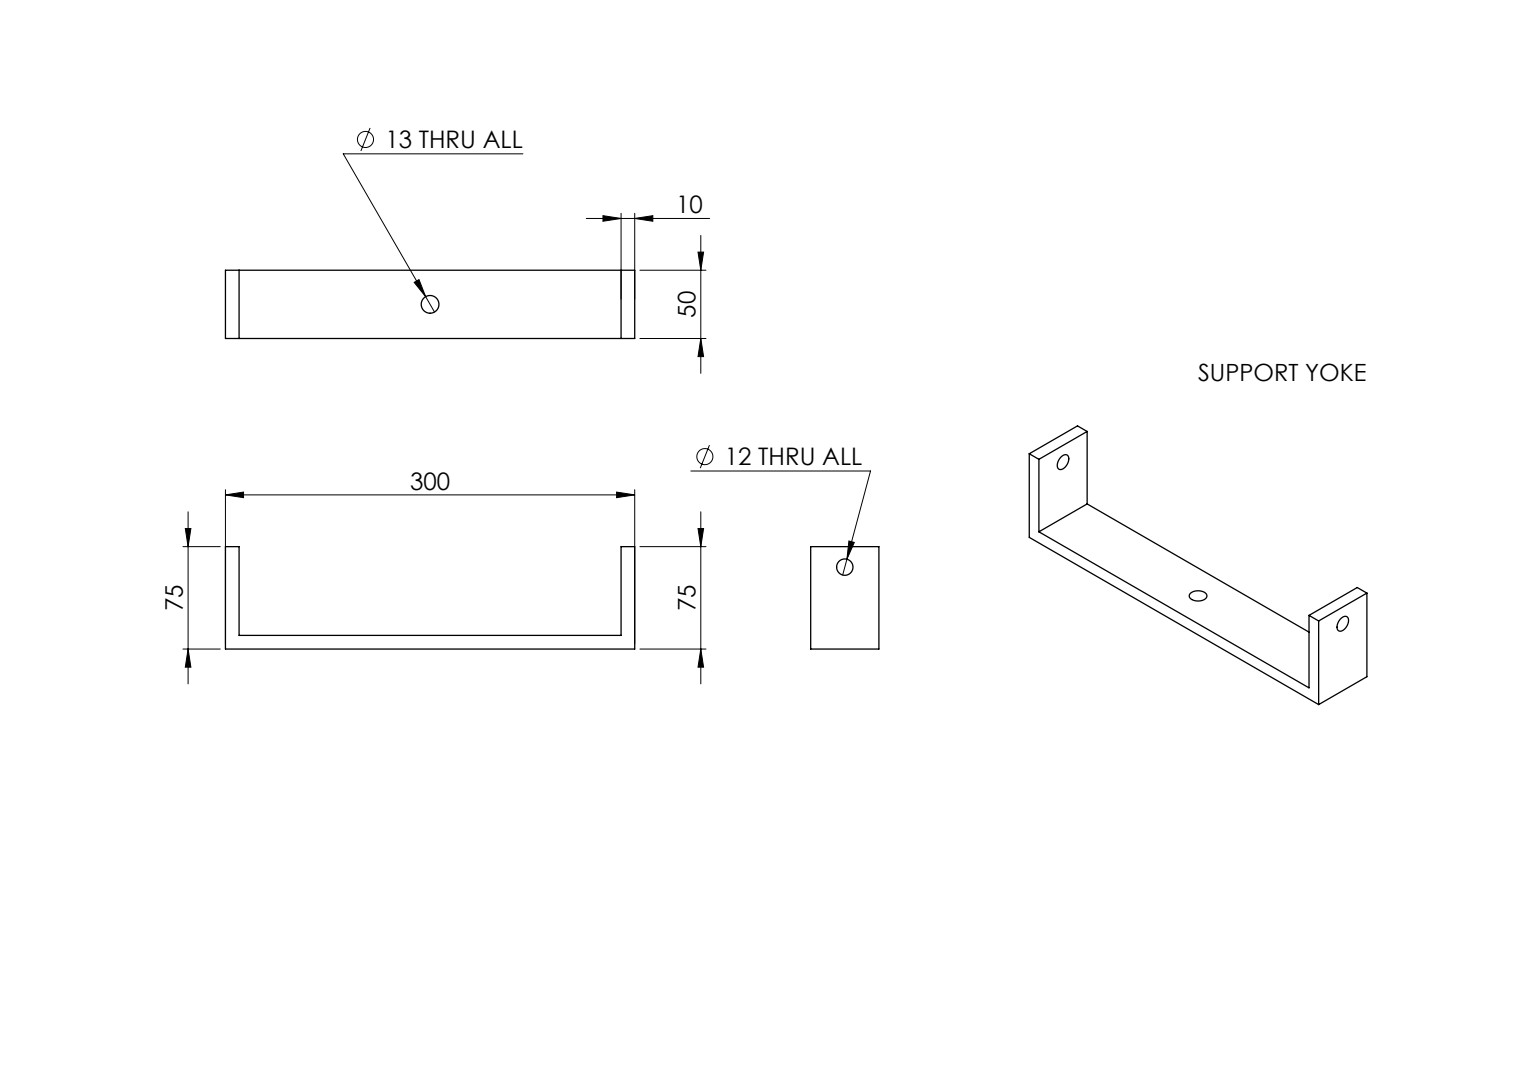
ISO-10303-21;
HEADER;
FILE_DESCRIPTION (('STEP AP214'),
    '1' );
FILE_NAME ('support yoke.step',
    '2026-10-22T16:49:52',
    ( '' ),
    ( '' ),
    'SwSTEP 2.0',
    'SolidWorks 2026',
    '' );
FILE_SCHEMA (( 'AUTOMOTIVE_DESIGN' ));
ENDSEC;

DATA;
#7=DIRECTION ( 'NONE',  ( 0.000000000000000000, 0.000000000000000000, -1.000000000000000000 ) ) ;
#8=DIRECTION ( 'NONE',  ( -1.000000000000000000, -0.000000000000000000, -0.000000000000000000 ) ) ;
#20=EDGE_LOOP ( 'NONE', ( #1630, #2560 ) ) ;
#23=ORIENTED_EDGE ( 'NONE', *, *, #198, .T. ) ;
#30=CARTESIAN_POINT ( 'NONE',  ( 150.0000000000000000, 810.0000000000000000, 25.00000000000000000 ) ) ;
#33=EDGE_LOOP ( 'NONE', ( #4983, #5227 ) ) ;
#50=CARTESIAN_POINT ( 'NONE',  ( -150.0000000000000000, 870.0000000000000000, 0.000000000000000000 ) ) ;
#67=STYLED_ITEM('',(#5412),#3780);
#72=CARTESIAN_POINT ( 'NONE',  ( -150.0000000000000000, 820.0000000000001137, 25.00000000000000000 ) ) ;
#79=EDGE_CURVE ( 'NONE', #3280, #3385, #2552, .T. ) ;
#80=EDGE_CURVE ( 'NONE', #4039, #3851, #2630, .T. ) ;
#99=ORIENTED_EDGE ( 'NONE', *, *, #4103, .T. ) ;
#103=DIRECTION ( 'NONE',  ( 1.000000000000000000, 0.000000000000000000, 0.000000000000000000 ) ) ;
#106=DIRECTION ( 'NONE',  ( 1.000000000000000000, 0.000000000000000000, 0.000000000000000000 ) ) ;
#112=PLANE ( 'NONE',  #5289 ) ;
#116=VECTOR ( 'NONE', #4178, 1000.000000000000000 ) ;
#148=VECTOR ( 'NONE', #4543, 1000.000000000000000 ) ;
#160=ORIENTED_EDGE ( 'NONE', *, *, #3298, .F. ) ;
#162=CARTESIAN_POINT ( 'NONE',  ( -150.0000000000000000, 870.0000000000000000, -6.000000000000006217 ) ) ;
#165=VERTEX_POINT ( 'NONE', #2690 ) ;
#191=DIRECTION ( 'NONE',  ( -0.000000000000000000, -1.000000000000000000, 0.000000000000000000 ) ) ;
#192=DIRECTION ( 'NONE',  ( -0.000000000000000000, 1.000000000000000000, -0.000000000000000000 ) ) ;
#197=ORIENTED_EDGE ( 'NONE', *, *, #3520, .F. ) ;
#198=EDGE_CURVE ( 'NONE', #3942, #4623, #5254, .T. ) ;
#206=EDGE_CURVE ( 'NONE', #3842, #5043, #2268, .T. ) ;
#238=ORIENTED_EDGE ( 'NONE', *, *, #1651, .F. ) ;
#247=CARTESIAN_POINT ( 'NONE',  ( 139.9999999999999716, 885.0000000000000000, -25.00000000000000000 ) ) ;
#249=ORIENTED_EDGE ( 'NONE', *, *, #342, .F. ) ;
#262=DIRECTION ( 'NONE',  ( 1.000000000000000000, 0.000000000000000000, 0.000000000000000000 ) ) ;
#280=CARTESIAN_POINT ( 'NONE',  ( 139.9999999999999716, 885.0000000000000000, 25.00000000000000000 ) ) ;
#286=EDGE_LOOP ( 'NONE', ( #1725, #726, #2392, #4939 ) ) ;
#300=VECTOR ( 'NONE', #2784, 1000.000000000000000 ) ;
#305=ADVANCED_FACE ( 'NONE', ( #1215, #3776 ), #1663, .T. ) ;
#330=DIRECTION ( 'NONE',  ( 0.000000000000000000, 0.000000000000000000, 1.000000000000000000 ) ) ;
#336=CIRCLE ( 'NONE', #2605, 5.999999999999894307 ) ;
#342=EDGE_CURVE ( 'NONE', #2324, #5253, #4160, .T. ) ;
#351=ORIENTED_EDGE ( 'NONE', *, *, #3520, .T. ) ;
#359=DIRECTION ( 'NONE',  ( 0.000000000000000000, 0.000000000000000000, -1.000000000000000000 ) ) ;
#371=DIRECTION ( 'NONE',  ( -0.000000000000000000, -0.000000000000000000, -1.000000000000000000 ) ) ;
#374=ORIENTED_EDGE ( 'NONE', *, *, #3449, .T. ) ;
#376=CARTESIAN_POINT ( 'NONE',  ( 139.9999999999999716, 820.0000000000001137, -25.00000000000000000 ) ) ;
#397=ORIENTED_EDGE ( 'NONE', *, *, #4687, .F. ) ;
#413=DIRECTION ( 'NONE',  ( 0.000000000000000000, 0.000000000000000000, 1.000000000000000000 ) ) ;
#427=ORIENTED_EDGE ( 'NONE', *, *, #4247, .F. ) ;
#436=CARTESIAN_POINT ( 'NONE',  ( -150.0000000000000000, 870.0000000000000000, -5.999999999999950262 ) ) ;
#443=PRODUCT ( 'support yoke', 'support yoke', '', ( #4465 ) ) ;
#451=ORIENTED_EDGE ( 'NONE', *, *, #2561, .F. ) ;
#455=ORIENTED_EDGE ( 'NONE', *, *, #4975, .F. ) ;
#457=VERTEX_POINT ( 'NONE', #162 ) ;
#485=( GEOMETRIC_REPRESENTATION_CONTEXT ( 3 ) GLOBAL_UNCERTAINTY_ASSIGNED_CONTEXT ( ( #3762 ) ) GLOBAL_UNIT_ASSIGNED_CONTEXT ( ( #4296, #3410, #1343 ) ) REPRESENTATION_CONTEXT ( 'NONE', 'WORKASPACE' ) );
#486=EDGE_LOOP ( 'NONE', ( #2087, #1135, #1675, #1922 ) ) ;
#489=DIRECTION ( 'NONE',  ( 1.000000000000000000, 0.000000000000000000, 0.000000000000000000 ) ) ;
#503=VERTEX_POINT ( 'NONE', #879 ) ;
#509=CIRCLE ( 'NONE', #2248, 6.499999999999999112 ) ;
#530=VECTOR ( 'NONE', #4346, 1000.000000000000000 ) ;
#535=EDGE_CURVE ( 'NONE', #4624, #5043, #1720, .T. ) ;
#556=PRESENTATION_STYLE_ASSIGNMENT (( #4250 ) ) ;
#570=CARTESIAN_POINT ( 'NONE',  ( -150.0000000000000000, 810.0000000000000000, -25.00000000000000000 ) ) ;
#583=CARTESIAN_POINT ( 'NONE',  ( 7.960204194457795477E-16, 810.0000000000000000, -6.499999999999999112 ) ) ;
#584=VECTOR ( 'NONE', #1682, 1000.000000000000000 ) ;
#586=LINE ( 'NONE', #5193, #5037 ) ;
#653=COLOUR_RGB ( '',0.8941176470588234615, 0.8941176470588234615, 0.8941176470588234615 ) ;
#654=ORIENTED_EDGE ( 'NONE', *, *, #80, .T. ) ;
#677=CARTESIAN_POINT ( 'NONE',  ( -150.0000000000000000, 810.0000000000000000, 25.00000000000000000 ) ) ;
#686=CARTESIAN_POINT ( 'NONE',  ( 150.0000000000000000, 885.0000000000000000, -25.00000000000000000 ) ) ;
#699=DIRECTION ( 'NONE',  ( 0.000000000000000000, 0.000000000000000000, 1.000000000000000000 ) ) ;
#705=ORIENTED_EDGE ( 'NONE', *, *, #198, .F. ) ;
#726=ORIENTED_EDGE ( 'NONE', *, *, #1041, .T. ) ;
#732=ORIENTED_EDGE ( 'NONE', *, *, #3637, .T. ) ;
#739=DIRECTION ( 'NONE',  ( 1.000000000000000000, -0.000000000000000000, -0.000000000000000000 ) ) ;
#766=DIRECTION ( 'NONE',  ( 0.000000000000000000, 0.000000000000000000, 1.000000000000000000 ) ) ;
#768=( GEOMETRIC_REPRESENTATION_CONTEXT ( 3 ) GLOBAL_UNCERTAINTY_ASSIGNED_CONTEXT ( ( #2886 ) ) GLOBAL_UNIT_ASSIGNED_CONTEXT ( ( #2204, #5209, #5150 ) ) REPRESENTATION_CONTEXT ( 'NONE', 'WORKASPACE' ) );
#769=DIRECTION ( 'NONE',  ( 1.000000000000000000, 0.000000000000000000, 0.000000000000000000 ) ) ;
#786=CARTESIAN_POINT ( 'NONE',  ( 139.9999999999999716, 885.0000000000000000, -25.00000000000000000 ) ) ;
#788=APPLICATION_CONTEXT ( 'automotive_design' ) ;
#800=LINE ( 'NONE', #247, #2779 ) ;
#814=EDGE_CURVE ( 'NONE', #3015, #3385, #852, .T. ) ;
#820=ORIENTED_EDGE ( 'NONE', *, *, #3637, .F. ) ;
#831=DIRECTION ( 'NONE',  ( -1.000000000000000000, 0.000000000000000000, 0.000000000000000000 ) ) ;
#836=CIRCLE ( 'NONE', #1178, 6.000000000000005329 ) ;
#837=ORIENTED_EDGE ( 'NONE', *, *, #4975, .T. ) ;
#843=CYLINDRICAL_SURFACE ( 'NONE', #2403, 6.500000000000000000 ) ;
#844=ORIENTED_EDGE ( 'NONE', *, *, #814, .F. ) ;
#849=VECTOR ( 'NONE', #191, 1000.000000000000000 ) ;
#850=VERTEX_POINT ( 'NONE', #5295 ) ;
#852=LINE ( 'NONE', #2846, #116 ) ;
#873=FACE_BOUND ( 'NONE', #4726, .T. ) ;
#875=ADVANCED_FACE ( 'NONE', ( #4126 ), #1205, .T. ) ;
#876=EDGE_CURVE ( 'NONE', #3385, #3280, #4904, .T. ) ;
#878=ORIENTED_EDGE ( 'NONE', *, *, #3994, .T. ) ;
#879=CARTESIAN_POINT ( 'NONE',  ( -150.0000000000000000, 810.0000000000000000, 25.00000000000000000 ) ) ;
#883=ORIENTED_EDGE ( 'NONE', *, *, #876, .F. ) ;
#891=DIRECTION ( 'NONE',  ( 0.000000000000000000, 0.000000000000000000, -1.000000000000000000 ) ) ;
#906=VECTOR ( 'NONE', #371, 1000.000000000000000 ) ;
#921=CIRCLE ( 'NONE', #2511, 5.999999999999894307 ) ;
#928=VECTOR ( 'NONE', #4600, 1000.000000000000000 ) ;
#950=DIRECTION ( 'NONE',  ( -1.000000000000000000, -0.000000000000000000, 0.000000000000000000 ) ) ;
#954=ORIENTED_EDGE ( 'NONE', *, *, #3467, .T. ) ;
#990=FILL_AREA_STYLE_COLOUR ( '', #653 ) ;
#992=EDGE_CURVE ( 'NONE', #1518, #3842, #1759, .T. ) ;
#998=AXIS2_PLACEMENT_3D ( 'NONE', #1508, #1083, #4072 ) ;
#1011=AXIS2_PLACEMENT_3D ( 'NONE', #2490, #2911, #4155 ) ;
#1017=LINE ( 'NONE', #4706, #2766 ) ;
#1027=ORIENTED_EDGE ( 'NONE', *, *, #2170, .F. ) ;
#1030=AXIS2_PLACEMENT_3D ( 'NONE', #4574, #3774, #413 ) ;
#1041=EDGE_CURVE ( 'NONE', #3303, #457, #1786, .T. ) ;
#1053=VECTOR ( 'NONE', #5134, 1000.000000000000000 ) ;
#1083=DIRECTION ( 'NONE',  ( 0.000000000000000000, 1.000000000000000000, 0.000000000000000000 ) ) ;
#1086=ORIENTED_EDGE ( 'NONE', *, *, #4012, .F. ) ;
#1098=DIRECTION ( 'NONE',  ( 0.000000000000000000, 0.000000000000000000, -1.000000000000000000 ) ) ;
#1102=EDGE_CURVE ( 'NONE', #4507, #850, #2281, .T. ) ;
#1108=ORIENTED_EDGE ( 'NONE', *, *, #79, .F. ) ;
#1127=CARTESIAN_POINT ( 'NONE',  ( 0.000000000000000000, 0.000000000000000000, 25.00000000000000000 ) ) ;
#1135=ORIENTED_EDGE ( 'NONE', *, *, #5039, .F. ) ;
#1137=EDGE_LOOP ( 'NONE', ( #2340, #4405, #654, #2970 ) ) ;
#1145=CARTESIAN_POINT ( 'NONE',  ( -139.9999999999999716, 810.0000000000000000, 25.00000000000000000 ) ) ;
#1155=CARTESIAN_POINT ( 'NONE',  ( -150.0000000000000000, 870.0000000000000000, 0.000000000000000000 ) ) ;
#1174=DIRECTION ( 'NONE',  ( 1.000000000000000000, 0.000000000000000000, -0.000000000000000000 ) ) ;
#1175=DIRECTION ( 'NONE',  ( 0.000000000000000000, 0.000000000000000000, 1.000000000000000000 ) ) ;
#1178=AXIS2_PLACEMENT_3D ( 'NONE', #50, #2614, #2635 ) ;
#1192=LINE ( 'NONE', #4977, #3207 ) ;
#1205=PLANE ( 'NONE',  #4466 ) ;
#1215=FACE_BOUND ( 'NONE', #3739, .T. ) ;
#1224=VERTEX_POINT ( 'NONE', #3925 ) ;
#1233=PLANE ( 'NONE',  #1011 ) ;
#1243=DIRECTION ( 'NONE',  ( -0.000000000000000000, -0.000000000000000000, -1.000000000000000000 ) ) ;
#1248=EDGE_CURVE ( 'NONE', #503, #3980, #2343, .T. ) ;
#1266=STYLED_ITEM ( 'NONE', ( #556 ), #5266 ) ;
#1268=ORIENTED_EDGE ( 'NONE', *, *, #1102, .F. ) ;
#1271=DIRECTION ( 'NONE',  ( -0.000000000000000000, -1.000000000000000000, -0.000000000000000000 ) ) ;
#1292=EDGE_CURVE ( 'NONE', #165, #2065, #2179, .T. ) ;
#1304=PLANE ( 'NONE',  #3654 ) ;
#1316=CARTESIAN_POINT ( 'NONE',  ( -150.0000000000000000, 870.0000000000000000, 0.000000000000000000 ) ) ;
#1323=LINE ( 'NONE', #4743, #2686 ) ;
#1325=AXIS2_PLACEMENT_3D ( 'NONE', #3342, #2525, #5331 ) ;
#1343=( NAMED_UNIT ( * ) SI_UNIT ( $, .STERADIAN. ) SOLID_ANGLE_UNIT ( ) );
#1345=MECHANICAL_DESIGN_GEOMETRIC_PRESENTATION_REPRESENTATION('',(#1266),#5013);
#1357=ORIENTED_EDGE ( 'NONE', *, *, #4166, .F. ) ;
#1359=CARTESIAN_POINT ( 'NONE',  ( -139.9999999999999716, 870.0000000000000000, 5.999999999999950262 ) ) ;
#1375=CARTESIAN_POINT ( 'NONE',  ( -139.9999999999999716, 820.0000000000001137, -25.00000000000000000 ) ) ;
#1379=CARTESIAN_POINT ( 'NONE',  ( -150.0000000000000000, 820.0000000000001137, -25.00000000000000000 ) ) ;
#1423=AXIS2_PLACEMENT_3D ( 'NONE', #1316, #2995, #2132 ) ;
#1428=EDGE_LOOP ( 'NONE', ( #3649, #4159, #2102, #844 ) ) ;
#1438=CARTESIAN_POINT ( 'NONE',  ( 150.0000000000000000, 885.0000000000000000, 25.00000000000000000 ) ) ;
#1444=VECTOR ( 'NONE', #2559, 1000.000000000000000 ) ;
#1464=ORIENTED_EDGE ( 'NONE', *, *, #1248, .F. ) ;
#1487=DIRECTION ( 'NONE',  ( 1.000000000000000000, 0.000000000000000000, 0.000000000000000000 ) ) ;
#1495=CARTESIAN_POINT ( 'NONE',  ( -150.0000000000000000, 870.0000000000000000, 0.000000000000000000 ) ) ;
#1498=FACE_OUTER_BOUND ( 'NONE', #1428, .T. ) ;
#1508=CARTESIAN_POINT ( 'NONE',  ( -150.0000000000000000, 810.0000000000000000, 25.00000000000000000 ) ) ;
#1518=VERTEX_POINT ( 'NONE', #2242 ) ;
#1564=ORIENTED_EDGE ( 'NONE', *, *, #2240, .T. ) ;
#1565=ORIENTED_EDGE ( 'NONE', *, *, #2151, .F. ) ;
#1577=LINE ( 'NONE', #4909, #4491 ) ;
#1584=EDGE_LOOP ( 'NONE', ( #1586, #820, #5321, #4418 ) ) ;
#1586=ORIENTED_EDGE ( 'NONE', *, *, #3467, .F. ) ;
#1595=ORIENTED_EDGE ( 'NONE', *, *, #2067, .F. ) ;
#1599=DIRECTION ( 'NONE',  ( 0.000000000000000000, 0.000000000000000000, 1.000000000000000000 ) ) ;
#1607=PRODUCT_DEFINITION_CONTEXT ( 'detailed design', #4664, 'design' ) ;
#1614=ORIENTED_EDGE ( 'NONE', *, *, #1292, .T. ) ;
#1620=SHAPE_REPRESENTATION ( 'support yoke', ( #4154 ), #485 ) ;
#1630=ORIENTED_EDGE ( 'NONE', *, *, #5039, .T. ) ;
#1635=FACE_OUTER_BOUND ( 'NONE', #1658, .T. ) ;
#1645=CARTESIAN_POINT ( 'NONE',  ( 150.0000000000000000, 810.0000000000000000, 25.00000000000000000 ) ) ;
#1651=EDGE_CURVE ( 'NONE', #3303, #3154, #3622, .T. ) ;
#1658=EDGE_LOOP ( 'NONE', ( #3325, #1595, #1614, #732 ) ) ;
#1663=PLANE ( 'NONE',  #1325 ) ;
#1675=ORIENTED_EDGE ( 'NONE', *, *, #814, .T. ) ;
#1682=DIRECTION ( 'NONE',  ( 0.000000000000000000, 1.000000000000000000, 0.000000000000000000 ) ) ;
#1707=CIRCLE ( 'NONE', #1423, 6.000000000000005329 ) ;
#1712=ORIENTED_EDGE ( 'NONE', *, *, #3751, .T. ) ;
#1720=LINE ( 'NONE', #5048, #4511 ) ;
#1725=ORIENTED_EDGE ( 'NONE', *, *, #3298, .T. ) ;
#1735=EDGE_LOOP ( 'NONE', ( #2336, #2444, #4389, #3297 ) ) ;
#1748=PLANE ( 'NONE',  #2875 ) ;
#1757=ORIENTED_EDGE ( 'NONE', *, *, #206, .T. ) ;
#1759=LINE ( 'NONE', #4692, #3954 ) ;
#1773=CARTESIAN_POINT ( 'NONE',  ( 139.9999999999999716, 885.0000000000000000, 25.00000000000000000 ) ) ;
#1779=ORIENTED_EDGE ( 'NONE', *, *, #4990, .F. ) ;
#1783=ORIENTED_EDGE ( 'NONE', *, *, #535, .F. ) ;
#1786=LINE ( 'NONE', #2093, #5353 ) ;
#1805=DIRECTION ( 'NONE',  ( -1.000000000000000000, -0.000000000000000000, 0.000000000000000000 ) ) ;
#1809=AXIS2_PLACEMENT_3D ( 'NONE', #3644, #4934, #1599 ) ;
#1822=CARTESIAN_POINT ( 'NONE',  ( -150.0000000000000000, 870.0000000000000000, 5.999999999999950262 ) ) ;
#1867=ORIENTED_EDGE ( 'NONE', *, *, #2240, .F. ) ;
#1882=LINE ( 'NONE', #2739, #4659 ) ;
#1922=ORIENTED_EDGE ( 'NONE', *, *, #876, .T. ) ;
#1925=CARTESIAN_POINT ( 'NONE',  ( -139.9999999999999716, 870.0000000000000000, 0.000000000000000000 ) ) ;
#1944=PLANE ( 'NONE',  #998 ) ;
#1945=AXIS2_PLACEMENT_3D ( 'NONE', #3613, #5271, #359 ) ;
#1953=CYLINDRICAL_SURFACE ( 'NONE', #1809, 5.999999999999950262 ) ;
#2015=DIRECTION ( 'NONE',  ( -1.000000000000000000, -0.000000000000000000, -0.000000000000000000 ) ) ;
#2024=EDGE_LOOP ( 'NONE', ( #1779, #5378, #5038, #249 ) ) ;
#2036=VERTEX_POINT ( 'NONE', #3689 ) ;
#2040=CYLINDRICAL_SURFACE ( 'NONE', #1030, 6.500000000000000000 ) ;
#2056=ADVANCED_FACE ( 'NONE', ( #2840 ), #843, .F. ) ;
#2065=VERTEX_POINT ( 'NONE', #2432 ) ;
#2067=EDGE_CURVE ( 'NONE', #165, #2036, #4515, .T. ) ;
#2070=ORIENTED_EDGE ( 'NONE', *, *, #2170, .T. ) ;
#2074=VECTOR ( 'NONE', #3618, 1000.000000000000000 ) ;
#2087=ORIENTED_EDGE ( 'NONE', *, *, #3943, .F. ) ;
#2088=ORIENTED_EDGE ( 'NONE', *, *, #1292, .F. ) ;
#2093=CARTESIAN_POINT ( 'NONE',  ( -150.0000000000000000, 870.0000000000000000, -5.999999999999950262 ) ) ;
#2102=ORIENTED_EDGE ( 'NONE', *, *, #79, .T. ) ;
#2126=FACE_OUTER_BOUND ( 'NONE', #1735, .T. ) ;
#2132=DIRECTION ( 'NONE',  ( 0.000000000000000000, 0.000000000000000000, 1.000000000000000000 ) ) ;
#2133=LINE ( 'NONE', #5002, #1444 ) ;
#2140=CARTESIAN_POINT ( 'NONE',  ( -150.0000000000000000, 810.0000000000000000, 25.00000000000000000 ) ) ;
#2142=CIRCLE ( 'NONE', #2860, 5.999999999999950262 ) ;
#2151=EDGE_CURVE ( 'NONE', #457, #3895, #836, .T. ) ;
#2170=EDGE_CURVE ( 'NONE', #165, #503, #3892, .T. ) ;
#2179=LINE ( 'NONE', #5123, #3715 ) ;
#2202=EDGE_LOOP ( 'NONE', ( #1268, #451, #4763, #1564 ) ) ;
#2204=( LENGTH_UNIT ( ) NAMED_UNIT ( * ) SI_UNIT ( .MILLI., .METRE. ) );
#2219=VECTOR ( 'NONE', #1271, 1000.000000000000000 ) ;
#2221=CIRCLE ( 'NONE', #2587, 6.499999999999999112 ) ;
#2228=CARTESIAN_POINT ( 'NONE',  ( -150.0000000000000000, 810.0000000000000000, -25.00000000000000000 ) ) ;
#2232=ORIENTED_EDGE ( 'NONE', *, *, #5241, .F. ) ;
#2240=EDGE_CURVE ( 'NONE', #5253, #850, #5182, .T. ) ;
#2242=CARTESIAN_POINT ( 'NONE',  ( 139.9999999999999716, 885.0000000000000000, 25.00000000000000000 ) ) ;
#2247=ORIENTED_EDGE ( 'NONE', *, *, #2067, .T. ) ;
#2248=AXIS2_PLACEMENT_3D ( 'NONE', #3992, #3161, #1175 ) ;
#2268=LINE ( 'NONE', #1438, #3844 ) ;
#2281=LINE ( 'NONE', #4377, #300 ) ;
#2296=LINE ( 'NONE', #3090, #849 ) ;
#2324=VERTEX_POINT ( 'NONE', #3507 ) ;
#2327=ADVANCED_FACE ( 'NONE', ( #1498 ), #3173, .F. ) ;
#2336=ORIENTED_EDGE ( 'NONE', *, *, #535, .T. ) ;
#2337=VECTOR ( 'NONE', #3898, 1000.000000000000000 ) ;
#2340=ORIENTED_EDGE ( 'NONE', *, *, #3767, .F. ) ;
#2343=LINE ( 'NONE', #677, #3085 ) ;
#2344=FACE_BOUND ( 'NONE', #33, .T. ) ;
#2386=LINE ( 'NONE', #280, #2074 ) ;
#2392=ORIENTED_EDGE ( 'NONE', *, *, #2151, .T. ) ;
#2403=AXIS2_PLACEMENT_3D ( 'NONE', #4485, #5343, #766 ) ;
#2405=CARTESIAN_POINT ( 'NONE',  ( 0.000000000000000000, 0.000000000000000000, -25.00000000000000000 ) ) ;
#2407=DIRECTION ( 'NONE',  ( 0.000000000000000000, 0.000000000000000000, -1.000000000000000000 ) ) ;
#2432=CARTESIAN_POINT ( 'NONE',  ( -139.9999999999999716, 885.0000000000000000, 25.00000000000000000 ) ) ;
#2434=CARTESIAN_POINT ( 'NONE',  ( 0.000000000000000000, 0.000000000000000000, 0.000000000000000000 ) ) ;
#2444=ORIENTED_EDGE ( 'NONE', *, *, #206, .F. ) ;
#2446=PLANE ( 'NONE',  #5377 ) ;
#2452=ORIENTED_EDGE ( 'NONE', *, *, #2562, .T. ) ;
#2455=CARTESIAN_POINT ( 'NONE',  ( -150.0000000000000000, 885.0000000000000000, 25.00000000000000000 ) ) ;
#2466=SHAPE_DEFINITION_REPRESENTATION ( #5021, #1620 ) ;
#2474=ORIENTED_EDGE ( 'NONE', *, *, #1651, .T. ) ;
#2489=FACE_OUTER_BOUND ( 'NONE', #5079, .T. ) ;
#2490=CARTESIAN_POINT ( 'NONE',  ( -150.0000000000000000, 885.0000000000000000, 25.00000000000000000 ) ) ;
#2511=AXIS2_PLACEMENT_3D ( 'NONE', #3251, #2015, #3226 ) ;
#2525=DIRECTION ( 'NONE',  ( 0.000000000000000000, 1.000000000000000000, 0.000000000000000000 ) ) ;
#2552=CIRCLE ( 'NONE', #2988, 5.999999999999950262 ) ;
#2558=CARTESIAN_POINT ( 'NONE',  ( 0.000000000000000000, 810.0000000000000000, 0.000000000000000000 ) ) ;
#2559=DIRECTION ( 'NONE',  ( -0.000000000000000000, -0.000000000000000000, -1.000000000000000000 ) ) ;
#2560=ORIENTED_EDGE ( 'NONE', *, *, #3359, .T. ) ;
#2561=EDGE_CURVE ( 'NONE', #2324, #4507, #2221, .T. ) ;
#2562=EDGE_CURVE ( 'NONE', #3895, #457, #1707, .T. ) ;
#2587=AXIS2_PLACEMENT_3D ( 'NONE', #2558, #4211, #2632 ) ;
#2605=AXIS2_PLACEMENT_3D ( 'NONE', #4464, #5350, #4414 ) ;
#2614=DIRECTION ( 'NONE',  ( -1.000000000000000000, -0.000000000000000000, -0.000000000000000000 ) ) ;
#2626=PLANE ( 'NONE',  #3396 ) ;
#2630=LINE ( 'NONE', #72, #1053 ) ;
#2632=DIRECTION ( 'NONE',  ( 0.000000000000000000, 0.000000000000000000, 1.000000000000000000 ) ) ;
#2635=DIRECTION ( 'NONE',  ( 0.000000000000000000, 0.000000000000000000, 1.000000000000000000 ) ) ;
#2637=EDGE_CURVE ( 'NONE', #850, #5253, #5278, .T. ) ;
#2666=SURFACE_STYLE_FILL_AREA ( #3509 ) ;
#2686=VECTOR ( 'NONE', #4009, 1000.000000000000000 ) ;
#2690=CARTESIAN_POINT ( 'NONE',  ( -150.0000000000000000, 885.0000000000000000, 25.00000000000000000 ) ) ;
#2699=SURFACE_SIDE_STYLE ('',( #2666 ) ) ;
#2724=ORIENTED_EDGE ( 'NONE', *, *, #1248, .T. ) ;
#2736=AXIS2_PLACEMENT_3D ( 'NONE', #3726, #4078, #330 ) ;
#2739=CARTESIAN_POINT ( 'NONE',  ( -150.0000000000000000, 810.0000000000000000, -25.00000000000000000 ) ) ;
#2745=CARTESIAN_POINT ( 'NONE',  ( -139.9999999999999716, 820.0000000000001137, 25.00000000000000000 ) ) ;
#2766=VECTOR ( 'NONE', #4317, 1000.000000000000000 ) ;
#2772=DIRECTION ( 'NONE',  ( -1.000000000000000000, -0.000000000000000000, -0.000000000000000000 ) ) ;
#2775=ADVANCED_FACE ( 'NONE', ( #3170 ), #4003, .F. ) ;
#2777=CARTESIAN_POINT ( 'NONE',  ( -150.0000000000000000, 870.0000000000000000, 0.000000000000000000 ) ) ;
#2778=DIRECTION ( 'NONE',  ( -0.000000000000000000, -1.000000000000000000, 0.000000000000000000 ) ) ;
#2779=VECTOR ( 'NONE', #1487, 1000.000000000000000 ) ;
#2784=DIRECTION ( 'NONE',  ( -0.000000000000000000, 1.000000000000000000, -0.000000000000000000 ) ) ;
#2789=FACE_BOUND ( 'NONE', #4125, .T. ) ;
#2816=CARTESIAN_POINT ( 'NONE',  ( 150.0000000000000000, 885.0000000000000000, 25.00000000000000000 ) ) ;
#2822=FACE_OUTER_BOUND ( 'NONE', #4974, .T. ) ;
#2827=ORIENTED_EDGE ( 'NONE', *, *, #1041, .F. ) ;
#2840=FACE_OUTER_BOUND ( 'NONE', #2202, .T. ) ;
#2846=CARTESIAN_POINT ( 'NONE',  ( -150.0000000000000000, 870.0000000000000000, 5.999999999999950262 ) ) ;
#2857=DIRECTION ( 'NONE',  ( -0.000000000000000000, -0.000000000000000000, -1.000000000000000000 ) ) ;
#2860=AXIS2_PLACEMENT_3D ( 'NONE', #1925, #739, #2407 ) ;
#2875=AXIS2_PLACEMENT_3D ( 'NONE', #1645, #831, #3758 ) ;
#2882=DIRECTION ( 'NONE',  ( -1.000000000000000000, 0.000000000000000000, -0.000000000000000000 ) ) ;
#2886=UNCERTAINTY_MEASURE_WITH_UNIT (LENGTH_MEASURE( 1.000000000000000082E-05 ), #2204, 'distance_accuracy_value', 'NONE');
#2910=CARTESIAN_POINT ( 'NONE',  ( -139.9999999999999716, 820.0000000000001137, 25.00000000000000000 ) ) ;
#2911=DIRECTION ( 'NONE',  ( 0.000000000000000000, 1.000000000000000000, 0.000000000000000000 ) ) ;
#2922=ORIENTED_EDGE ( 'NONE', *, *, #3767, .T. ) ;
#2936=LINE ( 'NONE', #30, #584 ) ;
#2949=EDGE_LOOP ( 'NONE', ( #2827, #2474, #1712, #2452 ) ) ;
#2962=LINE ( 'NONE', #3394, #928 ) ;
#2970=ORIENTED_EDGE ( 'NONE', *, *, #4395, .T. ) ;
#2988=AXIS2_PLACEMENT_3D ( 'NONE', #2994, #1805, #3913 ) ;
#2994=CARTESIAN_POINT ( 'NONE',  ( 139.9999999999999716, 870.0000000000000000, 0.000000000000000000 ) ) ;
#2995=DIRECTION ( 'NONE',  ( -1.000000000000000000, -0.000000000000000000, -0.000000000000000000 ) ) ;
#3013=FACE_BOUND ( 'NONE', #20, .T. ) ;
#3015=VERTEX_POINT ( 'NONE', #3401 ) ;
#3023=( NAMED_UNIT ( * ) SI_UNIT ( $, .STERADIAN. ) SOLID_ANGLE_UNIT ( ) );
#3035=LINE ( 'NONE', #1822, #3108 ) ;
#3067=DIRECTION ( 'NONE',  ( 0.000000000000000000, 1.000000000000000000, 0.000000000000000000 ) ) ;
#3085=VECTOR ( 'NONE', #262, 1000.000000000000000 ) ;
#3090=CARTESIAN_POINT ( 'NONE',  ( -139.9999999999999716, 810.0000000000000000, -25.00000000000000000 ) ) ;
#3096=CLOSED_SHELL ( 'NONE', ( #5140, #2327, #2775, #4770, #3514, #4826, #305, #3388, #3411, #4018, #5385, #3597, #875, #5096, #4619, #2056 ) ) ;
#3108=VECTOR ( 'NONE', #4263, 1000.000000000000000 ) ;
#3134=LINE ( 'NONE', #2228, #2337 ) ;
#3143=ORIENTED_EDGE ( 'NONE', *, *, #80, .F. ) ;
#3152=ORIENTED_EDGE ( 'NONE', *, *, #2562, .F. ) ;
#3154=VERTEX_POINT ( 'NONE', #1359 ) ;
#3161=DIRECTION ( 'NONE',  ( -0.000000000000000000, 1.000000000000000000, -0.000000000000000000 ) ) ;
#3170=FACE_OUTER_BOUND ( 'NONE', #286, .T. ) ;
#3173=CYLINDRICAL_SURFACE ( 'NONE', #5095, 5.999999999999950262 ) ;
#3195=CARTESIAN_POINT ( 'NONE',  ( 139.9999999999999716, 870.0000000000000000, 5.999999999999950262 ) ) ;
#3203=DIRECTION ( 'NONE',  ( -1.000000000000000000, 0.000000000000000000, -0.000000000000000000 ) ) ;
#3207=VECTOR ( 'NONE', #1243, 1000.000000000000000 ) ;
#3226=DIRECTION ( 'NONE',  ( 0.000000000000000000, 0.000000000000000000, 1.000000000000000000 ) ) ;
#3251=CARTESIAN_POINT ( 'NONE',  ( 150.0000000000000000, 870.0000000000000000, 0.000000000000000000 ) ) ;
#3280=VERTEX_POINT ( 'NONE', #5325 ) ;
#3297=ORIENTED_EDGE ( 'NONE', *, *, #4012, .T. ) ;
#3298=EDGE_CURVE ( 'NONE', #3154, #3303, #2142, .T. ) ;
#3303=VERTEX_POINT ( 'NONE', #4080 ) ;
#3314=LINE ( 'NONE', #436, #4937 ) ;
#3325=ORIENTED_EDGE ( 'NONE', *, *, #4103, .F. ) ;
#3342=CARTESIAN_POINT ( 'NONE',  ( -150.0000000000000000, 820.0000000000001137, 25.00000000000000000 ) ) ;
#3348=EDGE_LOOP ( 'NONE', ( #455, #397, #4195, #1757 ) ) ;
#3359=EDGE_CURVE ( 'NONE', #1224, #3015, #921, .T. ) ;
#3362=LINE ( 'NONE', #2910, #148 ) ;
#3371=CARTESIAN_POINT ( 'NONE',  ( 0.000000000000000000, 820.0000000000001137, 6.500000000000000000 ) ) ;
#3385=VERTEX_POINT ( 'NONE', #3195 ) ;
#3388=ADVANCED_FACE ( 'NONE', ( #2789, #4047 ), #4874, .T. ) ;
#3394=CARTESIAN_POINT ( 'NONE',  ( 150.0000000000000000, 810.0000000000000000, 25.00000000000000000 ) ) ;
#3396=AXIS2_PLACEMENT_3D ( 'NONE', #4361, #950, #4284 ) ;
#3401=CARTESIAN_POINT ( 'NONE',  ( 150.0000000000000000, 870.0000000000000000, 5.999999999999894307 ) ) ;
#3410=( NAMED_UNIT ( * ) PLANE_ANGLE_UNIT ( ) SI_UNIT ( $, .RADIAN. ) );
#3411=ADVANCED_FACE ( 'NONE', ( #1635 ), #1233, .T. ) ;
#3449=EDGE_CURVE ( 'NONE', #2036, #3744, #1882, .T. ) ;
#3456=DIRECTION ( 'NONE',  ( 0.000000000000000000, -0.000000000000000000, 1.000000000000000000 ) ) ;
#3467=EDGE_CURVE ( 'NONE', #4833, #5330, #2296, .T. ) ;
#3507=CARTESIAN_POINT ( 'NONE',  ( 0.000000000000000000, 810.0000000000000000, 6.499999999999999112 ) ) ;
#3509=FILL_AREA_STYLE ('',( #990 ) ) ;
#3514=ADVANCED_FACE ( 'NONE', ( #4392 ), #112, .T. ) ;
#3520=EDGE_CURVE ( 'NONE', #3851, #1518, #1017, .T. ) ;
#3551=LINE ( 'NONE', #1379, #5384 ) ;
#3554=VECTOR ( 'NONE', #4468, 1000.000000000000000 ) ;
#3597=ADVANCED_FACE ( 'NONE', ( #2822 ), #2446, .F. ) ;
#3613=CARTESIAN_POINT ( 'NONE',  ( -139.9999999999999716, 870.0000000000000000, 0.000000000000000000 ) ) ;
#3618=DIRECTION ( 'NONE',  ( -0.000000000000000000, -0.000000000000000000, -1.000000000000000000 ) ) ;
#3622=CIRCLE ( 'NONE', #1945, 5.999999999999950262 ) ;
#3637=EDGE_CURVE ( 'NONE', #2065, #4833, #1577, .T. ) ;
#3644=CARTESIAN_POINT ( 'NONE',  ( -150.0000000000000000, 870.0000000000000000, 0.000000000000000000 ) ) ;
#3649=ORIENTED_EDGE ( 'NONE', *, *, #3359, .F. ) ;
#3654=AXIS2_PLACEMENT_3D ( 'NONE', #4620, #4153, #891 ) ;
#3689=CARTESIAN_POINT ( 'NONE',  ( -150.0000000000000000, 885.0000000000000000, -25.00000000000000000 ) ) ;
#3715=VECTOR ( 'NONE', #103, 1000.000000000000000 ) ;
#3726=CARTESIAN_POINT ( 'NONE',  ( 139.9999999999999716, 870.0000000000000000, 0.000000000000000000 ) ) ;
#3739=EDGE_LOOP ( 'NONE', ( #1867, #4810 ) ) ;
#3744=VERTEX_POINT ( 'NONE', #570 ) ;
#3751=EDGE_CURVE ( 'NONE', #3154, #3895, #3035, .T. ) ;
#3758=DIRECTION ( 'NONE',  ( 0.000000000000000000, 0.000000000000000000, 1.000000000000000000 ) ) ;
#3762=UNCERTAINTY_MEASURE_WITH_UNIT (LENGTH_MEASURE( 1.000000000000000082E-05 ), #4296, 'distance_accuracy_value', 'NONE');
#3767=EDGE_CURVE ( 'NONE', #5330, #3942, #3551, .T. ) ;
#3774=DIRECTION ( 'NONE',  ( -0.000000000000000000, 1.000000000000000000, -0.000000000000000000 ) ) ;
#3776=FACE_OUTER_BOUND ( 'NONE', #1137, .T. ) ;
#3780=MANIFOLD_SOLID_BREP ( 'M12 Clearance Hole1', #3096 ) ;
#3796=CARTESIAN_POINT ( 'NONE',  ( 150.0000000000000000, 810.0000000000000000, 25.00000000000000000 ) ) ;
#3800=AXIS2_PLACEMENT_3D ( 'NONE', #5163, #5192, #3973 ) ;
#3842=VERTEX_POINT ( 'NONE', #2816 ) ;
#3844=VECTOR ( 'NONE', #5217, 1000.000000000000000 ) ;
#3851=VERTEX_POINT ( 'NONE', #5262 ) ;
#3880=CARTESIAN_POINT ( 'NONE',  ( -139.9999999999999716, 885.0000000000000000, -25.00000000000000000 ) ) ;
#3892=LINE ( 'NONE', #2140, #2219 ) ;
#3895=VERTEX_POINT ( 'NONE', #4900 ) ;
#3898=DIRECTION ( 'NONE',  ( 1.000000000000000000, 0.000000000000000000, 0.000000000000000000 ) ) ;
#3911=ORIENTED_EDGE ( 'NONE', *, *, #4247, .T. ) ;
#3913=DIRECTION ( 'NONE',  ( 0.000000000000000000, 0.000000000000000000, 1.000000000000000000 ) ) ;
#3925=CARTESIAN_POINT ( 'NONE',  ( 150.0000000000000000, 870.0000000000000000, -5.999999999999894307 ) ) ;
#3939=DIRECTION ( 'NONE',  ( -0.000000000000000000, -1.000000000000000000, -0.000000000000000000 ) ) ;
#3942=VERTEX_POINT ( 'NONE', #376 ) ;
#3943=EDGE_CURVE ( 'NONE', #1224, #3280, #3314, .T. ) ;
#3954=VECTOR ( 'NONE', #489, 1000.000000000000000 ) ;
#3966=DIRECTION ( 'NONE',  ( 0.000000000000000000, 0.000000000000000000, 1.000000000000000000 ) ) ;
#3973=DIRECTION ( 'NONE',  ( 0.000000000000000000, 0.000000000000000000, 1.000000000000000000 ) ) ;
#3980=VERTEX_POINT ( 'NONE', #3796 ) ;
#3985=FACE_OUTER_BOUND ( 'NONE', #4365, .T. ) ;
#3992=CARTESIAN_POINT ( 'NONE',  ( 0.000000000000000000, 810.0000000000000000, 0.000000000000000000 ) ) ;
#3994=EDGE_CURVE ( 'NONE', #3980, #3842, #2936, .T. ) ;
#3999=EDGE_CURVE ( 'NONE', #4039, #5330, #3362, .T. ) ;
#4003=CYLINDRICAL_SURFACE ( 'NONE', #4323, 5.999999999999950262 ) ;
#4009=DIRECTION ( 'NONE',  ( 1.000000000000000000, 0.000000000000000000, 0.000000000000000000 ) ) ;
#4012=EDGE_CURVE ( 'NONE', #3980, #4624, #2962, .T. ) ;
#4018=ADVANCED_FACE ( 'NONE', ( #873, #2489 ), #1304, .F. ) ;
#4039=VERTEX_POINT ( 'NONE', #2745 ) ;
#4047=FACE_OUTER_BOUND ( 'NONE', #1584, .T. ) ;
#4048=FACE_OUTER_BOUND ( 'NONE', #2949, .T. ) ;
#4060=CYLINDRICAL_SURFACE ( 'NONE', #4666, 5.999999999999950262 ) ;
#4072=DIRECTION ( 'NONE',  ( 0.000000000000000000, -0.000000000000000000, 1.000000000000000000 ) ) ;
#4078=DIRECTION ( 'NONE',  ( -1.000000000000000000, -0.000000000000000000, 0.000000000000000000 ) ) ;
#4080=CARTESIAN_POINT ( 'NONE',  ( -139.9999999999999716, 870.0000000000000000, -5.999999999999950262 ) ) ;
#4103=EDGE_CURVE ( 'NONE', #2036, #4833, #1323, .T. ) ;
#4119=EDGE_LOOP ( 'NONE', ( #705, #4272, #351, #5336 ) ) ;
#4125=EDGE_LOOP ( 'NONE', ( #160, #238 ) ) ;
#4126=FACE_OUTER_BOUND ( 'NONE', #5128, .T. ) ;
#4153=DIRECTION ( 'NONE',  ( 1.000000000000000000, 0.000000000000000000, 0.000000000000000000 ) ) ;
#4154=AXIS2_PLACEMENT_3D ( 'NONE', #2434, #5290, #769 ) ;
#4155=DIRECTION ( 'NONE',  ( 0.000000000000000000, -0.000000000000000000, 1.000000000000000000 ) ) ;
#4159=ORIENTED_EDGE ( 'NONE', *, *, #3943, .T. ) ;
#4160=LINE ( 'NONE', #3371, #3554 ) ;
#4166=EDGE_CURVE ( 'NONE', #2065, #4039, #586, .T. ) ;
#4178=DIRECTION ( 'NONE',  ( -1.000000000000000000, -0.000000000000000000, -0.000000000000000000 ) ) ;
#4195=ORIENTED_EDGE ( 'NONE', *, *, #992, .T. ) ;
#4200=FACE_OUTER_BOUND ( 'NONE', #2024, .T. ) ;
#4211=DIRECTION ( 'NONE',  ( -0.000000000000000000, 1.000000000000000000, -0.000000000000000000 ) ) ;
#4247=EDGE_CURVE ( 'NONE', #503, #3744, #1192, .T. ) ;
#4250=SURFACE_STYLE_USAGE ( .BOTH. , #2699 ) ;
#4263=DIRECTION ( 'NONE',  ( -1.000000000000000000, -0.000000000000000000, -0.000000000000000000 ) ) ;
#4272=ORIENTED_EDGE ( 'NONE', *, *, #4395, .F. ) ;
#4284=DIRECTION ( 'NONE',  ( 0.000000000000000000, 0.000000000000000000, 1.000000000000000000 ) ) ;
#4296=( LENGTH_UNIT ( ) NAMED_UNIT ( * ) SI_UNIT ( .MILLI., .METRE. ) );
#4299=ORIENTED_EDGE ( 'NONE', *, *, #992, .F. ) ;
#4316=CARTESIAN_POINT ( 'NONE',  ( 139.9999999999999716, 810.0000000000000000, -25.00000000000000000 ) ) ;
#4317=DIRECTION ( 'NONE',  ( -0.000000000000000000, 1.000000000000000000, 0.000000000000000000 ) ) ;
#4318=PRODUCT_DEFINITION_FORMATION_WITH_SPECIFIED_SOURCE ( 'ANY', '', #443, .NOT_KNOWN. ) ;
#4321=AXIS2_PLACEMENT_3D ( 'NONE', #4348, #192, #3966 ) ;
#4323=AXIS2_PLACEMENT_3D ( 'NONE', #1495, #2772, #4823 ) ;
#4325=( LENGTH_UNIT ( ) NAMED_UNIT ( * ) SI_UNIT ( .MILLI., .METRE. ) );
#4346=DIRECTION ( 'NONE',  ( -0.000000000000000000, 1.000000000000000000, 0.000000000000000000 ) ) ;
#4348=CARTESIAN_POINT ( 'NONE',  ( 0.000000000000000000, 820.0000000000001137, 0.000000000000000000 ) ) ;
#4361=CARTESIAN_POINT ( 'NONE',  ( 139.9999999999999716, 810.0000000000000000, 25.00000000000000000 ) ) ;
#4365=EDGE_LOOP ( 'NONE', ( #4453, #1086, #1464, #3911 ) ) ;
#4377=CARTESIAN_POINT ( 'NONE',  ( 7.960204194457795477E-16, 820.0000000000001137, -6.500000000000000000 ) ) ;
#4389=ORIENTED_EDGE ( 'NONE', *, *, #3994, .F. ) ;
#4392=FACE_OUTER_BOUND ( 'NONE', #3348, .T. ) ;
#4395=EDGE_CURVE ( 'NONE', #3851, #3942, #2133, .T. ) ;
#4405=ORIENTED_EDGE ( 'NONE', *, *, #3999, .F. ) ;
#4414=DIRECTION ( 'NONE',  ( 0.000000000000000000, 0.000000000000000000, 1.000000000000000000 ) ) ;
#4418=ORIENTED_EDGE ( 'NONE', *, *, #3999, .T. ) ;
#4425=DIRECTION ( 'NONE',  ( -1.000000000000000000, -0.000000000000000000, -0.000000000000000000 ) ) ;
#4448=FACE_OUTER_BOUND ( 'NONE', #486, .T. ) ;
#4453=ORIENTED_EDGE ( 'NONE', *, *, #5241, .T. ) ;
#4464=CARTESIAN_POINT ( 'NONE',  ( 150.0000000000000000, 870.0000000000000000, 0.000000000000000000 ) ) ;
#4465=PRODUCT_CONTEXT ( 'NONE', #788, 'mechanical' ) ;
#4466=AXIS2_PLACEMENT_3D ( 'NONE', #2405, #7, #2882 ) ;
#4468=DIRECTION ( 'NONE',  ( -0.000000000000000000, 1.000000000000000000, -0.000000000000000000 ) ) ;
#4485=CARTESIAN_POINT ( 'NONE',  ( 0.000000000000000000, 820.0000000000001137, 0.000000000000000000 ) ) ;
#4491=VECTOR ( 'NONE', #2857, 1000.000000000000000 ) ;
#4507=VERTEX_POINT ( 'NONE', #583 ) ;
#4511=VECTOR ( 'NONE', #4625, 1000.000000000000000 ) ;
#4515=LINE ( 'NONE', #2455, #906 ) ;
#4543=DIRECTION ( 'NONE',  ( -0.000000000000000000, -0.000000000000000000, -1.000000000000000000 ) ) ;
#4574=CARTESIAN_POINT ( 'NONE',  ( 0.000000000000000000, 820.0000000000001137, 0.000000000000000000 ) ) ;
#4600=DIRECTION ( 'NONE',  ( -0.000000000000000000, -0.000000000000000000, -1.000000000000000000 ) ) ;
#4619=ADVANCED_FACE ( 'NONE', ( #4448 ), #4060, .F. ) ;
#4620=CARTESIAN_POINT ( 'NONE',  ( -150.0000000000000000, 810.0000000000000000, 25.00000000000000000 ) ) ;
#4623=VERTEX_POINT ( 'NONE', #786 ) ;
#4624=VERTEX_POINT ( 'NONE', #4943 ) ;
#4625=DIRECTION ( 'NONE',  ( 0.000000000000000000, 1.000000000000000000, 0.000000000000000000 ) ) ;
#4638=SHAPE_REPRESENTATION_RELATIONSHIP ( 'NONE' , 'NONE' ,  #1620, #5266 ) ;
#4659=VECTOR ( 'NONE', #3939, 1000.000000000000000 ) ;
#4661=UNCERTAINTY_MEASURE_WITH_UNIT (LENGTH_MEASURE( 1.000000000000000082E-05 ), #4325, 'distance_accuracy_value', 'NONE');
#4664=APPLICATION_CONTEXT ( 'automotive_design' ) ;
#4666=AXIS2_PLACEMENT_3D ( 'NONE', #1155, #4855, #5358 ) ;
#4667=( NAMED_UNIT ( * ) PLANE_ANGLE_UNIT ( ) SI_UNIT ( $, .RADIAN. ) );
#4670=DIRECTION ( 'NONE',  ( -1.000000000000000000, -0.000000000000000000, -0.000000000000000000 ) ) ;
#4687=EDGE_CURVE ( 'NONE', #1518, #4623, #2386, .T. ) ;
#4692=CARTESIAN_POINT ( 'NONE',  ( 139.9999999999999716, 885.0000000000000000, 25.00000000000000000 ) ) ;
#4706=CARTESIAN_POINT ( 'NONE',  ( 139.9999999999999716, 810.0000000000000000, 25.00000000000000000 ) ) ;
#4718=CARTESIAN_POINT ( 'NONE',  ( 0.000000000000000000, 820.0000000000001137, 6.500000000000000888 ) ) ;
#4726=EDGE_LOOP ( 'NONE', ( #3152, #1565 ) ) ;
#4727=FACE_BOUND ( 'NONE', #4870, .T. ) ;
#4743=CARTESIAN_POINT ( 'NONE',  ( -150.0000000000000000, 885.0000000000000000, -25.00000000000000000 ) ) ;
#4745=MECHANICAL_DESIGN_GEOMETRIC_PRESENTATION_REPRESENTATION('',(#67),#768);
#4763=ORIENTED_EDGE ( 'NONE', *, *, #342, .T. ) ;
#4770=ADVANCED_FACE ( 'NONE', ( #3013, #2126 ), #1748, .F. ) ;
#4788=FACE_OUTER_BOUND ( 'NONE', #4119, .T. ) ;
#4810=ORIENTED_EDGE ( 'NONE', *, *, #2637, .F. ) ;
#4823=DIRECTION ( 'NONE',  ( 0.000000000000000000, 0.000000000000000000, 1.000000000000000000 ) ) ;
#4826=ADVANCED_FACE ( 'NONE', ( #4727, #4788 ), #2626, .T. ) ;
#4833=VERTEX_POINT ( 'NONE', #3880 ) ;
#4855=DIRECTION ( 'NONE',  ( -1.000000000000000000, -0.000000000000000000, -0.000000000000000000 ) ) ;
#4870=EDGE_LOOP ( 'NONE', ( #883, #1108 ) ) ;
#4874=PLANE ( 'NONE',  #5191 ) ;
#4900=CARTESIAN_POINT ( 'NONE',  ( -150.0000000000000000, 870.0000000000000000, 6.000000000000005329 ) ) ;
#4904=CIRCLE ( 'NONE', #2736, 5.999999999999950262 ) ;
#4909=CARTESIAN_POINT ( 'NONE',  ( -139.9999999999999716, 885.0000000000000000, 25.00000000000000000 ) ) ;
#4925=ORIENTED_EDGE ( 'NONE', *, *, #3449, .F. ) ;
#4934=DIRECTION ( 'NONE',  ( -1.000000000000000000, -0.000000000000000000, -0.000000000000000000 ) ) ;
#4937=VECTOR ( 'NONE', #8, 1000.000000000000000 ) ;
#4939=ORIENTED_EDGE ( 'NONE', *, *, #3751, .F. ) ;
#4943=CARTESIAN_POINT ( 'NONE',  ( 150.0000000000000000, 810.0000000000000000, -25.00000000000000000 ) ) ;
#4974=EDGE_LOOP ( 'NONE', ( #878, #4299, #197, #3143, #1357, #2088, #2070, #2724 ) ) ;
#4975=EDGE_CURVE ( 'NONE', #4623, #5043, #800, .T. ) ;
#4977=CARTESIAN_POINT ( 'NONE',  ( -150.0000000000000000, 810.0000000000000000, 25.00000000000000000 ) ) ;
#4983=ORIENTED_EDGE ( 'NONE', *, *, #2561, .T. ) ;
#4990=EDGE_CURVE ( 'NONE', #4507, #2324, #509, .T. ) ;
#5002=CARTESIAN_POINT ( 'NONE',  ( 139.9999999999999716, 820.0000000000001137, 25.00000000000000000 ) ) ;
#5013=( GEOMETRIC_REPRESENTATION_CONTEXT ( 3 ) GLOBAL_UNCERTAINTY_ASSIGNED_CONTEXT ( ( #4661 ) ) GLOBAL_UNIT_ASSIGNED_CONTEXT ( ( #4325, #4667, #3023 ) ) REPRESENTATION_CONTEXT ( 'NONE', 'WORKASPACE' ) );
#5021=PRODUCT_DEFINITION_SHAPE ( 'NONE', 'NONE',  #5255 ) ;
#5037=VECTOR ( 'NONE', #2778, 1000.000000000000000 ) ;
#5038=ORIENTED_EDGE ( 'NONE', *, *, #2637, .T. ) ;
#5039=EDGE_CURVE ( 'NONE', #3015, #1224, #336, .T. ) ;
#5043=VERTEX_POINT ( 'NONE', #686 ) ;
#5048=CARTESIAN_POINT ( 'NONE',  ( 150.0000000000000000, 810.0000000000000000, -25.00000000000000000 ) ) ;
#5079=EDGE_LOOP ( 'NONE', ( #374, #427, #1027, #2247 ) ) ;
#5095=AXIS2_PLACEMENT_3D ( 'NONE', #2777, #4425, #699 ) ;
#5096=ADVANCED_FACE ( 'NONE', ( #4048 ), #1953, .F. ) ;
#5123=CARTESIAN_POINT ( 'NONE',  ( -150.0000000000000000, 885.0000000000000000, 25.00000000000000000 ) ) ;
#5128=EDGE_LOOP ( 'NONE', ( #1783, #2232, #4925, #99, #954, #2922, #23, #837 ) ) ;
#5134=DIRECTION ( 'NONE',  ( 1.000000000000000000, 0.000000000000000000, 0.000000000000000000 ) ) ;
#5140=ADVANCED_FACE ( 'NONE', ( #4200 ), #2040, .F. ) ;
#5150=( NAMED_UNIT ( * ) SI_UNIT ( $, .STERADIAN. ) SOLID_ANGLE_UNIT ( ) );
#5163=CARTESIAN_POINT ( 'NONE',  ( 0.000000000000000000, 820.0000000000001137, 0.000000000000000000 ) ) ;
#5182=CIRCLE ( 'NONE', #3800, 6.500000000000000888 ) ;
#5191=AXIS2_PLACEMENT_3D ( 'NONE', #1145, #1174, #5381 ) ;
#5192=DIRECTION ( 'NONE',  ( -0.000000000000000000, 1.000000000000000000, -0.000000000000000000 ) ) ;
#5193=CARTESIAN_POINT ( 'NONE',  ( -139.9999999999999716, 810.0000000000000000, 25.00000000000000000 ) ) ;
#5209=( NAMED_UNIT ( * ) PLANE_ANGLE_UNIT ( ) SI_UNIT ( $, .RADIAN. ) );
#5217=DIRECTION ( 'NONE',  ( -0.000000000000000000, -0.000000000000000000, -1.000000000000000000 ) ) ;
#5227=ORIENTED_EDGE ( 'NONE', *, *, #4990, .T. ) ;
#5241=EDGE_CURVE ( 'NONE', #3744, #4624, #3134, .T. ) ;
#5253=VERTEX_POINT ( 'NONE', #4718 ) ;
#5254=LINE ( 'NONE', #4316, #530 ) ;
#5255=PRODUCT_DEFINITION ( 'UNKNOWN', '', #4318, #1607 ) ;
#5262=CARTESIAN_POINT ( 'NONE',  ( 139.9999999999999716, 820.0000000000001137, 25.00000000000000000 ) ) ;
#5266=ADVANCED_BREP_SHAPE_REPRESENTATION ( '', ( #3780, #4154 ), #485 ) ;
#5271=DIRECTION ( 'NONE',  ( 1.000000000000000000, -0.000000000000000000, -0.000000000000000000 ) ) ;
#5278=CIRCLE ( 'NONE', #4321, 6.500000000000000888 ) ;
#5289=AXIS2_PLACEMENT_3D ( 'NONE', #1773, #3067, #3456 ) ;
#5290=DIRECTION ( 'NONE',  ( 0.000000000000000000, 0.000000000000000000, 1.000000000000000000 ) ) ;
#5295=CARTESIAN_POINT ( 'NONE',  ( 7.960204194457797449E-16, 820.0000000000001137, -6.500000000000001776 ) ) ;
#5321=ORIENTED_EDGE ( 'NONE', *, *, #4166, .T. ) ;
#5325=CARTESIAN_POINT ( 'NONE',  ( 139.9999999999999716, 870.0000000000000000, -5.999999999999950262 ) ) ;
#5330=VERTEX_POINT ( 'NONE', #1375 ) ;
#5331=DIRECTION ( 'NONE',  ( 0.000000000000000000, -0.000000000000000000, 1.000000000000000000 ) ) ;
#5336=ORIENTED_EDGE ( 'NONE', *, *, #4687, .T. ) ;
#5343=DIRECTION ( 'NONE',  ( -0.000000000000000000, 1.000000000000000000, -0.000000000000000000 ) ) ;
#5350=DIRECTION ( 'NONE',  ( -1.000000000000000000, -0.000000000000000000, -0.000000000000000000 ) ) ;
#5353=VECTOR ( 'NONE', #4670, 1000.000000000000000 ) ;
#5358=DIRECTION ( 'NONE',  ( 0.000000000000000000, 0.000000000000000000, 1.000000000000000000 ) ) ;
#5377=AXIS2_PLACEMENT_3D ( 'NONE', #1127, #1098, #3203 ) ;
#5378=ORIENTED_EDGE ( 'NONE', *, *, #1102, .T. ) ;
#5381=DIRECTION ( 'NONE',  ( -0.000000000000000000, 0.000000000000000000, -1.000000000000000000 ) ) ;
#5384=VECTOR ( 'NONE', #106, 1000.000000000000000 ) ;
#5385=ADVANCED_FACE ( 'NONE', ( #2344, #3985 ), #1944, .F. ) ;
#5406=COLOUR_RGB('Light Blue',0.38,0.62,0.78);
#5407=FILL_AREA_STYLE_COLOUR('',#5406);
#5408=FILL_AREA_STYLE('',(#5407));
#5409=SURFACE_STYLE_FILL_AREA(#5408);
#5410=SURFACE_SIDE_STYLE('',(#5409));
#5411=SURFACE_STYLE_USAGE(.BOTH.,#5410);
#5412=PRESENTATION_STYLE_ASSIGNMENT((#5411));
ENDSEC;
END-ISO-10303-21;
